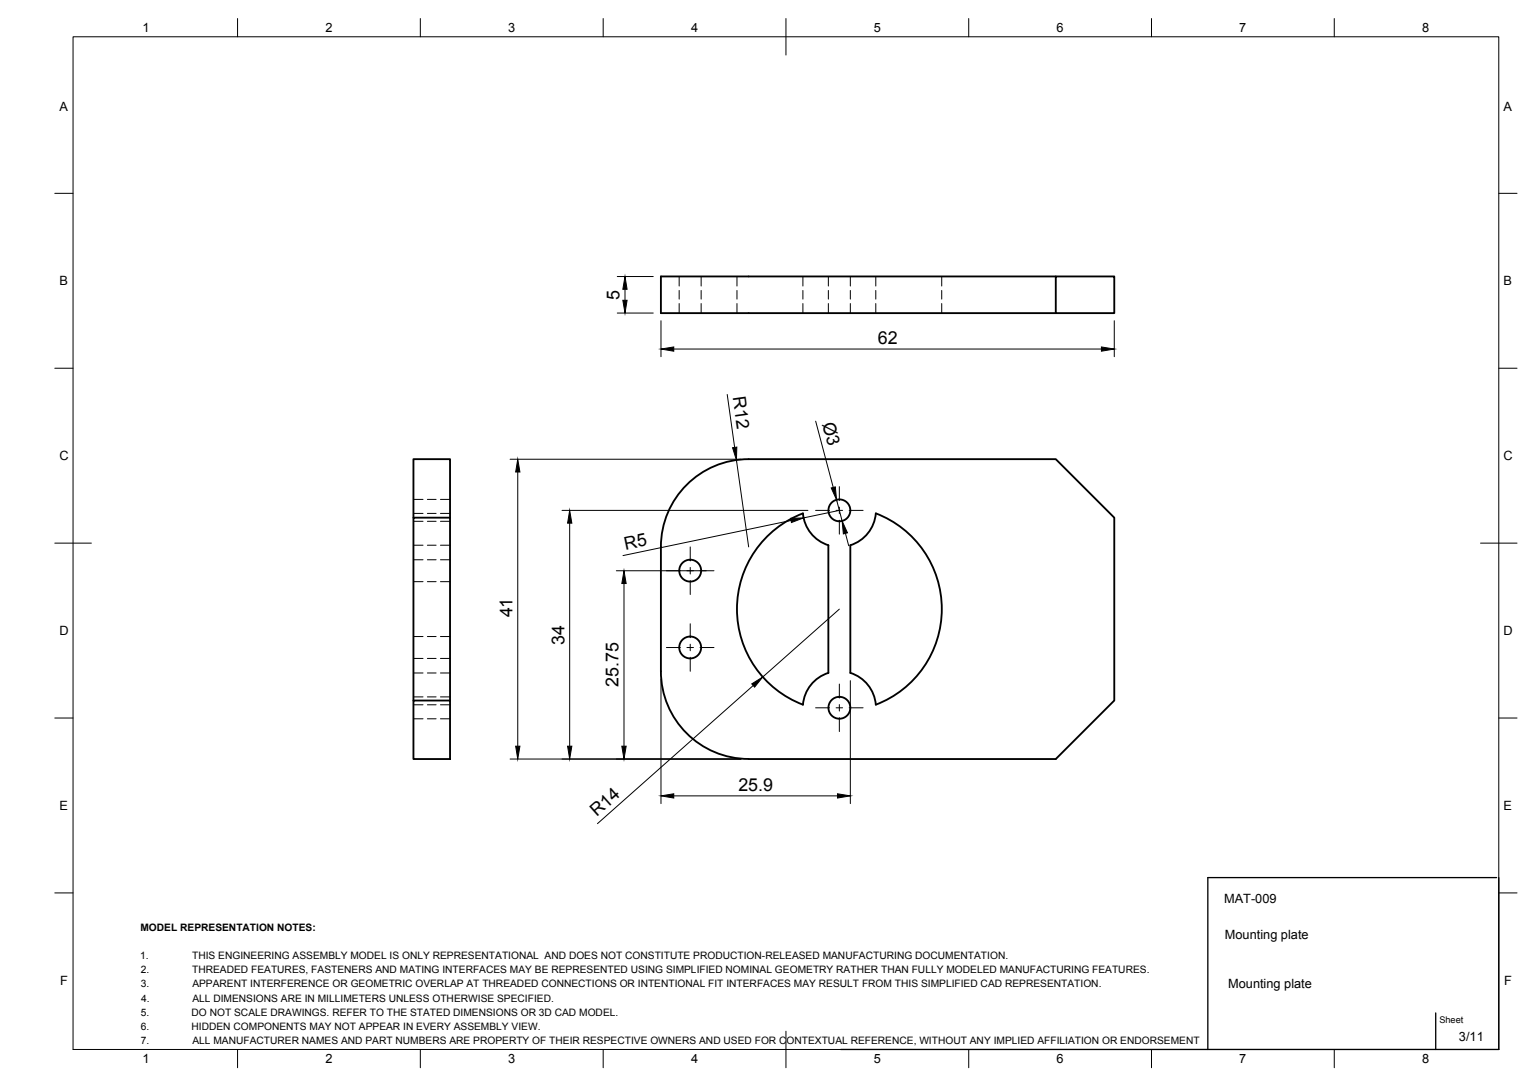
ISO-10303-21;
HEADER;
/* Generated by software containing ST-Developer
 * from STEP Tools, Inc. (www.steptools.com) 
 */

FILE_DESCRIPTION(
/* description */ ('STEP AP214'),
/* implementation_level */ '2;1');

FILE_NAME(
/* name */ 'Mounting Plate.step',
/* time_stamp */ '2026-11-14T05:43:09-08:00',
/* author */ (''),
/* organization */ (''),
/* preprocessor_version */ 'ST-DEVELOPER v20.2',
/* originating_system */ 'Autodesk Translation Framework v15.17.0.0',
/* authorisation */ '');

FILE_SCHEMA (('AUTOMOTIVE_DESIGN { 1 0 10303 214 3 1 1 }'));
ENDSEC;

DATA;
#10=MECHANICAL_DESIGN_GEOMETRIC_PRESENTATION_REPRESENTATION('',(#146),#11933);
#128=SHAPE_REPRESENTATION_RELATIONSHIP('SRR','None',#11988,#137);
#137=ADVANCED_BREP_SHAPE_REPRESENTATION('',(#155),#11924);
#146=STYLED_ITEM('',(#12042),#155);
#155=MANIFOLD_SOLID_BREP('Body1',#6643);
#164=FACE_BOUND('',#692,.T.);
#165=FACE_BOUND('',#693,.T.);
#166=FACE_BOUND('',#694,.T.);
#167=FACE_BOUND('',#695,.T.);
#168=FACE_BOUND('',#696,.T.);
#169=FACE_BOUND('',#697,.T.);
#170=FACE_BOUND('',#699,.T.);
#171=FACE_BOUND('',#700,.T.);
#172=FACE_BOUND('',#701,.T.);
#173=FACE_BOUND('',#702,.T.);
#174=FACE_BOUND('',#703,.T.);
#175=FACE_BOUND('',#704,.T.);
#209=PLANE('',#6766);
#210=PLANE('',#6767);
#211=PLANE('',#6768);
#212=PLANE('',#6769);
#213=PLANE('',#6770);
#214=PLANE('',#6777);
#215=PLANE('',#6787);
#216=PLANE('',#6791);
#217=PLANE('',#6792);
#218=PLANE('',#6795);
#319=FACE_OUTER_BOUND('',#673,.T.);
#320=FACE_OUTER_BOUND('',#674,.T.);
#321=FACE_OUTER_BOUND('',#675,.T.);
#322=FACE_OUTER_BOUND('',#676,.T.);
#323=FACE_OUTER_BOUND('',#677,.T.);
#324=FACE_OUTER_BOUND('',#678,.T.);
#325=FACE_OUTER_BOUND('',#679,.T.);
#326=FACE_OUTER_BOUND('',#680,.T.);
#327=FACE_OUTER_BOUND('',#681,.T.);
#328=FACE_OUTER_BOUND('',#682,.T.);
#329=FACE_OUTER_BOUND('',#683,.T.);
#330=FACE_OUTER_BOUND('',#684,.T.);
#331=FACE_OUTER_BOUND('',#685,.T.);
#332=FACE_OUTER_BOUND('',#686,.T.);
#333=FACE_OUTER_BOUND('',#687,.T.);
#334=FACE_OUTER_BOUND('',#688,.T.);
#335=FACE_OUTER_BOUND('',#689,.T.);
#336=FACE_OUTER_BOUND('',#690,.T.);
#337=FACE_OUTER_BOUND('',#691,.T.);
#338=FACE_OUTER_BOUND('',#698,.T.);
#339=FACE_OUTER_BOUND('',#705,.T.);
#340=FACE_OUTER_BOUND('',#706,.T.);
#673=EDGE_LOOP('',(#4112,#4113,#4114,#4115));
#674=EDGE_LOOP('',(#4116,#4117,#4118,#4119));
#675=EDGE_LOOP('',(#4120,#4121,#4122,#4123));
#676=EDGE_LOOP('',(#4124,#4125,#4126,#4127));
#677=EDGE_LOOP('',(#4128,#4129,#4130,#4131));
#678=EDGE_LOOP('',(#4132,#4133,#4134,#4135));
#679=EDGE_LOOP('',(#4136,#4137,#4138,#4139));
#680=EDGE_LOOP('',(#4140,#4141,#4142,#4143));
#681=EDGE_LOOP('',(#4144,#4145,#4146,#4147));
#682=EDGE_LOOP('',(#4148,#4149,#4150,#4151));
#683=EDGE_LOOP('',(#4152,#4153,#4154,#4155));
#684=EDGE_LOOP('',(#4156,#4157,#4158,#4159));
#685=EDGE_LOOP('',(#4160,#4161,#4162,#4163));
#686=EDGE_LOOP('',(#4164,#4165,#4166,#4167));
#687=EDGE_LOOP('',(#4168,#4169,#4170,#4171));
#688=EDGE_LOOP('',(#4172,#4173,#4174,#4175));
#689=EDGE_LOOP('',(#4176,#4177,#4178,#4179));
#690=EDGE_LOOP('',(#4180,#4181,#4182,#4183));
#691=EDGE_LOOP('',(#4184,#4185,#4186,#4187,#4188,#4189,#4190,#4191));
#692=EDGE_LOOP('',(#4192));
#693=EDGE_LOOP('',(#4193));
#694=EDGE_LOOP('',(#4194));
#695=EDGE_LOOP('',(#4195));
#696=EDGE_LOOP('',(#4196,#4197,#4198,#4199));
#697=EDGE_LOOP('',(#4200,#4201,#4202,#4203));
#698=EDGE_LOOP('',(#4204,#4205,#4206,#4207,#4208,#4209,#4210,#4211));
#699=EDGE_LOOP('',(#4212));
#700=EDGE_LOOP('',(#4213));
#701=EDGE_LOOP('',(#4214));
#702=EDGE_LOOP('',(#4215));
#703=EDGE_LOOP('',(#4216,#4217,#4218,#4219));
#704=EDGE_LOOP('',(#4220,#4221,#4222,#4223));
#705=EDGE_LOOP('',(#4224,#4225,#4226,#4227));
#706=EDGE_LOOP('',(#4228,#4229,#4230,#4231));
#1072=LINE('',#9914,#1534);
#1073=LINE('',#9920,#1535);
#1074=LINE('',#9926,#1536);
#1075=LINE('',#9932,#1537);
#1076=LINE('',#9937,#1538);
#1077=LINE('',#9939,#1539);
#1078=LINE('',#9941,#1540);
#1079=LINE('',#9942,#1541);
#1080=LINE('',#9945,#1542);
#1081=LINE('',#9947,#1543);
#1082=LINE('',#9948,#1544);
#1083=LINE('',#9951,#1545);
#1084=LINE('',#9953,#1546);
#1085=LINE('',#9954,#1547);
#1086=LINE('',#9957,#1548);
#1087=LINE('',#9959,#1549);
#1088=LINE('',#9960,#1550);
#1089=LINE('',#9964,#1551);
#1090=LINE('',#9966,#1552);
#1091=LINE('',#9968,#1553);
#1092=LINE('',#9969,#1554);
#1093=LINE('',#9975,#1555);
#1094=LINE('',#9978,#1556);
#1095=LINE('',#9983,#1557);
#1096=LINE('',#9987,#1558);
#1097=LINE('',#9989,#1559);
#1098=LINE('',#9990,#1560);
#1099=LINE('',#9996,#1561);
#1100=LINE('',#9999,#1562);
#1101=LINE('',#10004,#1563);
#1102=LINE('',#10010,#1564);
#1103=LINE('',#10014,#1565);
#1104=LINE('',#10016,#1566);
#1105=LINE('',#10017,#1567);
#1106=LINE('',#10022,#1568);
#1107=LINE('',#10023,#1569);
#1534=VECTOR('',#7658,1.5);
#1535=VECTOR('',#7665,1.5);
#1536=VECTOR('',#7672,1.5);
#1537=VECTOR('',#7679,1.5);
#1538=VECTOR('',#7684,1000.);
#1539=VECTOR('',#7685,1000.);
#1540=VECTOR('',#7686,1000.);
#1541=VECTOR('',#7687,1000.);
#1542=VECTOR('',#7690,1000.);
#1543=VECTOR('',#7691,1000.);
#1544=VECTOR('',#7692,1000.);
#1545=VECTOR('',#7695,1000.);
#1546=VECTOR('',#7696,1000.);
#1547=VECTOR('',#7697,1000.);
#1548=VECTOR('',#7700,1000.);
#1549=VECTOR('',#7701,1000.);
#1550=VECTOR('',#7702,1000.);
#1551=VECTOR('',#7705,1000.);
#1552=VECTOR('',#7706,1000.);
#1553=VECTOR('',#7707,1000.);
#1554=VECTOR('',#7708,1000.);
#1555=VECTOR('',#7713,1000.);
#1556=VECTOR('',#7716,1000.);
#1557=VECTOR('',#7721,1000.);
#1558=VECTOR('',#7726,1000.);
#1559=VECTOR('',#7727,1000.);
#1560=VECTOR('',#7728,1000.);
#1561=VECTOR('',#7733,1000.);
#1562=VECTOR('',#7736,1000.);
#1563=VECTOR('',#7741,1000.);
#1564=VECTOR('',#7748,1000.);
#1565=VECTOR('',#7753,1000.);
#1566=VECTOR('',#7754,1000.);
#1567=VECTOR('',#7755,1000.);
#1568=VECTOR('',#7764,1000.);
#1569=VECTOR('',#7765,1000.);
#1996=CIRCLE('',#6755,1.5);
#1997=CIRCLE('',#6756,1.5);
#1998=CIRCLE('',#6758,1.5);
#1999=CIRCLE('',#6759,1.5);
#2000=CIRCLE('',#6761,1.5);
#2001=CIRCLE('',#6762,1.5);
#2002=CIRCLE('',#6764,1.5);
#2003=CIRCLE('',#6765,1.5);
#2004=CIRCLE('',#6772,14.);
#2005=CIRCLE('',#6773,14.);
#2006=CIRCLE('',#6775,5.);
#2007=CIRCLE('',#6776,5.);
#2008=CIRCLE('',#6779,5.);
#2009=CIRCLE('',#6780,5.);
#2010=CIRCLE('',#6782,14.);
#2011=CIRCLE('',#6783,14.);
#2012=CIRCLE('',#6785,5.);
#2013=CIRCLE('',#6786,5.);
#2014=CIRCLE('',#6789,5.);
#2015=CIRCLE('',#6790,5.);
#2016=CIRCLE('',#6793,12.);
#2017=CIRCLE('',#6794,12.);
#2018=CIRCLE('',#6796,12.);
#2019=CIRCLE('',#6797,12.);
#2501=VERTEX_POINT('',#9911);
#2502=VERTEX_POINT('',#9913);
#2503=VERTEX_POINT('',#9917);
#2504=VERTEX_POINT('',#9919);
#2505=VERTEX_POINT('',#9923);
#2506=VERTEX_POINT('',#9925);
#2507=VERTEX_POINT('',#9929);
#2508=VERTEX_POINT('',#9931);
#2509=VERTEX_POINT('',#9935);
#2510=VERTEX_POINT('',#9936);
#2511=VERTEX_POINT('',#9938);
#2512=VERTEX_POINT('',#9940);
#2513=VERTEX_POINT('',#9944);
#2514=VERTEX_POINT('',#9946);
#2515=VERTEX_POINT('',#9950);
#2516=VERTEX_POINT('',#9952);
#2517=VERTEX_POINT('',#9956);
#2518=VERTEX_POINT('',#9958);
#2519=VERTEX_POINT('',#9962);
#2520=VERTEX_POINT('',#9963);
#2521=VERTEX_POINT('',#9965);
#2522=VERTEX_POINT('',#9967);
#2523=VERTEX_POINT('',#9971);
#2524=VERTEX_POINT('',#9972);
#2525=VERTEX_POINT('',#9974);
#2526=VERTEX_POINT('',#9976);
#2527=VERTEX_POINT('',#9980);
#2528=VERTEX_POINT('',#9982);
#2529=VERTEX_POINT('',#9986);
#2530=VERTEX_POINT('',#9988);
#2531=VERTEX_POINT('',#9992);
#2532=VERTEX_POINT('',#9993);
#2533=VERTEX_POINT('',#9995);
#2534=VERTEX_POINT('',#9997);
#2535=VERTEX_POINT('',#10001);
#2536=VERTEX_POINT('',#10003);
#2537=VERTEX_POINT('',#10007);
#2538=VERTEX_POINT('',#10009);
#2539=VERTEX_POINT('',#10013);
#2540=VERTEX_POINT('',#10015);
#3145=EDGE_CURVE('',#2501,#2501,#1996,.T.);
#3146=EDGE_CURVE('',#2501,#2502,#1072,.T.);
#3147=EDGE_CURVE('',#2502,#2502,#1997,.T.);
#3148=EDGE_CURVE('',#2503,#2503,#1998,.T.);
#3149=EDGE_CURVE('',#2503,#2504,#1073,.T.);
#3150=EDGE_CURVE('',#2504,#2504,#1999,.T.);
#3151=EDGE_CURVE('',#2505,#2505,#2000,.T.);
#3152=EDGE_CURVE('',#2505,#2506,#1074,.T.);
#3153=EDGE_CURVE('',#2506,#2506,#2001,.T.);
#3154=EDGE_CURVE('',#2507,#2507,#2002,.T.);
#3155=EDGE_CURVE('',#2507,#2508,#1075,.T.);
#3156=EDGE_CURVE('',#2508,#2508,#2003,.T.);
#3157=EDGE_CURVE('',#2509,#2510,#1076,.T.);
#3158=EDGE_CURVE('',#2511,#2510,#1077,.T.);
#3159=EDGE_CURVE('',#2512,#2511,#1078,.T.);
#3160=EDGE_CURVE('',#2512,#2509,#1079,.T.);
#3161=EDGE_CURVE('',#2510,#2513,#1080,.T.);
#3162=EDGE_CURVE('',#2514,#2513,#1081,.T.);
#3163=EDGE_CURVE('',#2511,#2514,#1082,.T.);
#3164=EDGE_CURVE('',#2515,#2513,#1083,.T.);
#3165=EDGE_CURVE('',#2516,#2515,#1084,.T.);
#3166=EDGE_CURVE('',#2516,#2514,#1085,.T.);
#3167=EDGE_CURVE('',#2515,#2517,#1086,.T.);
#3168=EDGE_CURVE('',#2517,#2518,#1087,.T.);
#3169=EDGE_CURVE('',#2516,#2518,#1088,.T.);
#3170=EDGE_CURVE('',#2519,#2520,#1089,.T.);
#3171=EDGE_CURVE('',#2519,#2521,#1090,.T.);
#3172=EDGE_CURVE('',#2521,#2522,#1091,.T.);
#3173=EDGE_CURVE('',#2522,#2520,#1092,.T.);
#3174=EDGE_CURVE('',#2523,#2524,#2004,.T.);
#3175=EDGE_CURVE('',#2525,#2523,#1093,.T.);
#3176=EDGE_CURVE('',#2525,#2526,#2005,.T.);
#3177=EDGE_CURVE('',#2526,#2524,#1094,.T.);
#3178=EDGE_CURVE('',#2527,#2523,#2006,.T.);
#3179=EDGE_CURVE('',#2528,#2527,#1095,.T.);
#3180=EDGE_CURVE('',#2528,#2525,#2007,.T.);
#3181=EDGE_CURVE('',#2529,#2527,#1096,.T.);
#3182=EDGE_CURVE('',#2530,#2529,#1097,.T.);
#3183=EDGE_CURVE('',#2530,#2528,#1098,.T.);
#3184=EDGE_CURVE('',#2531,#2532,#2008,.T.);
#3185=EDGE_CURVE('',#2533,#2531,#1099,.T.);
#3186=EDGE_CURVE('',#2533,#2534,#2009,.T.);
#3187=EDGE_CURVE('',#2534,#2532,#1100,.T.);
#3188=EDGE_CURVE('',#2535,#2531,#2010,.T.);
#3189=EDGE_CURVE('',#2536,#2535,#1101,.T.);
#3190=EDGE_CURVE('',#2536,#2533,#2011,.T.);
#3191=EDGE_CURVE('',#2535,#2537,#2012,.T.);
#3192=EDGE_CURVE('',#2538,#2537,#1102,.T.);
#3193=EDGE_CURVE('',#2536,#2538,#2013,.T.);
#3194=EDGE_CURVE('',#2539,#2512,#1103,.T.);
#3195=EDGE_CURVE('',#2539,#2540,#1104,.T.);
#3196=EDGE_CURVE('',#2540,#2509,#1105,.T.);
#3197=EDGE_CURVE('',#2529,#2524,#2014,.T.);
#3198=EDGE_CURVE('',#2530,#2526,#2015,.T.);
#3199=EDGE_CURVE('',#2537,#2532,#1106,.T.);
#3200=EDGE_CURVE('',#2538,#2534,#1107,.T.);
#3201=EDGE_CURVE('',#2518,#2519,#2016,.T.);
#3202=EDGE_CURVE('',#2520,#2539,#2017,.T.);
#3203=EDGE_CURVE('',#2521,#2517,#2018,.T.);
#3204=EDGE_CURVE('',#2540,#2522,#2019,.T.);
#4112=ORIENTED_EDGE('',*,*,#3145,.F.);
#4113=ORIENTED_EDGE('',*,*,#3146,.T.);
#4114=ORIENTED_EDGE('',*,*,#3147,.T.);
#4115=ORIENTED_EDGE('',*,*,#3146,.F.);
#4116=ORIENTED_EDGE('',*,*,#3148,.T.);
#4117=ORIENTED_EDGE('',*,*,#3149,.T.);
#4118=ORIENTED_EDGE('',*,*,#3150,.F.);
#4119=ORIENTED_EDGE('',*,*,#3149,.F.);
#4120=ORIENTED_EDGE('',*,*,#3151,.T.);
#4121=ORIENTED_EDGE('',*,*,#3152,.T.);
#4122=ORIENTED_EDGE('',*,*,#3153,.F.);
#4123=ORIENTED_EDGE('',*,*,#3152,.F.);
#4124=ORIENTED_EDGE('',*,*,#3154,.T.);
#4125=ORIENTED_EDGE('',*,*,#3155,.T.);
#4126=ORIENTED_EDGE('',*,*,#3156,.F.);
#4127=ORIENTED_EDGE('',*,*,#3155,.F.);
#4128=ORIENTED_EDGE('',*,*,#3157,.T.);
#4129=ORIENTED_EDGE('',*,*,#3158,.F.);
#4130=ORIENTED_EDGE('',*,*,#3159,.F.);
#4131=ORIENTED_EDGE('',*,*,#3160,.T.);
#4132=ORIENTED_EDGE('',*,*,#3161,.T.);
#4133=ORIENTED_EDGE('',*,*,#3162,.F.);
#4134=ORIENTED_EDGE('',*,*,#3163,.F.);
#4135=ORIENTED_EDGE('',*,*,#3158,.T.);
#4136=ORIENTED_EDGE('',*,*,#3164,.F.);
#4137=ORIENTED_EDGE('',*,*,#3165,.F.);
#4138=ORIENTED_EDGE('',*,*,#3166,.T.);
#4139=ORIENTED_EDGE('',*,*,#3162,.T.);
#4140=ORIENTED_EDGE('',*,*,#3167,.T.);
#4141=ORIENTED_EDGE('',*,*,#3168,.T.);
#4142=ORIENTED_EDGE('',*,*,#3169,.F.);
#4143=ORIENTED_EDGE('',*,*,#3165,.T.);
#4144=ORIENTED_EDGE('',*,*,#3170,.F.);
#4145=ORIENTED_EDGE('',*,*,#3171,.T.);
#4146=ORIENTED_EDGE('',*,*,#3172,.T.);
#4147=ORIENTED_EDGE('',*,*,#3173,.T.);
#4148=ORIENTED_EDGE('',*,*,#3174,.F.);
#4149=ORIENTED_EDGE('',*,*,#3175,.F.);
#4150=ORIENTED_EDGE('',*,*,#3176,.T.);
#4151=ORIENTED_EDGE('',*,*,#3177,.T.);
#4152=ORIENTED_EDGE('',*,*,#3178,.F.);
#4153=ORIENTED_EDGE('',*,*,#3179,.F.);
#4154=ORIENTED_EDGE('',*,*,#3180,.T.);
#4155=ORIENTED_EDGE('',*,*,#3175,.T.);
#4156=ORIENTED_EDGE('',*,*,#3181,.F.);
#4157=ORIENTED_EDGE('',*,*,#3182,.F.);
#4158=ORIENTED_EDGE('',*,*,#3183,.T.);
#4159=ORIENTED_EDGE('',*,*,#3179,.T.);
#4160=ORIENTED_EDGE('',*,*,#3184,.F.);
#4161=ORIENTED_EDGE('',*,*,#3185,.F.);
#4162=ORIENTED_EDGE('',*,*,#3186,.T.);
#4163=ORIENTED_EDGE('',*,*,#3187,.T.);
#4164=ORIENTED_EDGE('',*,*,#3188,.F.);
#4165=ORIENTED_EDGE('',*,*,#3189,.F.);
#4166=ORIENTED_EDGE('',*,*,#3190,.T.);
#4167=ORIENTED_EDGE('',*,*,#3185,.T.);
#4168=ORIENTED_EDGE('',*,*,#3191,.T.);
#4169=ORIENTED_EDGE('',*,*,#3192,.F.);
#4170=ORIENTED_EDGE('',*,*,#3193,.F.);
#4171=ORIENTED_EDGE('',*,*,#3189,.T.);
#4172=ORIENTED_EDGE('',*,*,#3194,.F.);
#4173=ORIENTED_EDGE('',*,*,#3195,.T.);
#4174=ORIENTED_EDGE('',*,*,#3196,.T.);
#4175=ORIENTED_EDGE('',*,*,#3160,.F.);
#4176=ORIENTED_EDGE('',*,*,#3197,.T.);
#4177=ORIENTED_EDGE('',*,*,#3177,.F.);
#4178=ORIENTED_EDGE('',*,*,#3198,.F.);
#4179=ORIENTED_EDGE('',*,*,#3182,.T.);
#4180=ORIENTED_EDGE('',*,*,#3199,.T.);
#4181=ORIENTED_EDGE('',*,*,#3187,.F.);
#4182=ORIENTED_EDGE('',*,*,#3200,.F.);
#4183=ORIENTED_EDGE('',*,*,#3192,.T.);
#4184=ORIENTED_EDGE('',*,*,#3169,.T.);
#4185=ORIENTED_EDGE('',*,*,#3201,.T.);
#4186=ORIENTED_EDGE('',*,*,#3170,.T.);
#4187=ORIENTED_EDGE('',*,*,#3202,.T.);
#4188=ORIENTED_EDGE('',*,*,#3194,.T.);
#4189=ORIENTED_EDGE('',*,*,#3159,.T.);
#4190=ORIENTED_EDGE('',*,*,#3163,.T.);
#4191=ORIENTED_EDGE('',*,*,#3166,.F.);
#4192=ORIENTED_EDGE('',*,*,#3154,.F.);
#4193=ORIENTED_EDGE('',*,*,#3145,.T.);
#4194=ORIENTED_EDGE('',*,*,#3148,.F.);
#4195=ORIENTED_EDGE('',*,*,#3151,.F.);
#4196=ORIENTED_EDGE('',*,*,#3186,.F.);
#4197=ORIENTED_EDGE('',*,*,#3190,.F.);
#4198=ORIENTED_EDGE('',*,*,#3193,.T.);
#4199=ORIENTED_EDGE('',*,*,#3200,.T.);
#4200=ORIENTED_EDGE('',*,*,#3176,.F.);
#4201=ORIENTED_EDGE('',*,*,#3180,.F.);
#4202=ORIENTED_EDGE('',*,*,#3183,.F.);
#4203=ORIENTED_EDGE('',*,*,#3198,.T.);
#4204=ORIENTED_EDGE('',*,*,#3172,.F.);
#4205=ORIENTED_EDGE('',*,*,#3203,.T.);
#4206=ORIENTED_EDGE('',*,*,#3167,.F.);
#4207=ORIENTED_EDGE('',*,*,#3164,.T.);
#4208=ORIENTED_EDGE('',*,*,#3161,.F.);
#4209=ORIENTED_EDGE('',*,*,#3157,.F.);
#4210=ORIENTED_EDGE('',*,*,#3196,.F.);
#4211=ORIENTED_EDGE('',*,*,#3204,.T.);
#4212=ORIENTED_EDGE('',*,*,#3156,.T.);
#4213=ORIENTED_EDGE('',*,*,#3147,.F.);
#4214=ORIENTED_EDGE('',*,*,#3150,.T.);
#4215=ORIENTED_EDGE('',*,*,#3153,.T.);
#4216=ORIENTED_EDGE('',*,*,#3184,.T.);
#4217=ORIENTED_EDGE('',*,*,#3199,.F.);
#4218=ORIENTED_EDGE('',*,*,#3191,.F.);
#4219=ORIENTED_EDGE('',*,*,#3188,.T.);
#4220=ORIENTED_EDGE('',*,*,#3174,.T.);
#4221=ORIENTED_EDGE('',*,*,#3197,.F.);
#4222=ORIENTED_EDGE('',*,*,#3181,.T.);
#4223=ORIENTED_EDGE('',*,*,#3178,.T.);
#4224=ORIENTED_EDGE('',*,*,#3201,.F.);
#4225=ORIENTED_EDGE('',*,*,#3168,.F.);
#4226=ORIENTED_EDGE('',*,*,#3203,.F.);
#4227=ORIENTED_EDGE('',*,*,#3171,.F.);
#4228=ORIENTED_EDGE('',*,*,#3202,.F.);
#4229=ORIENTED_EDGE('',*,*,#3173,.F.);
#4230=ORIENTED_EDGE('',*,*,#3204,.F.);
#4231=ORIENTED_EDGE('',*,*,#3195,.F.);
#6046=CYLINDRICAL_SURFACE('',#6754,1.5);
#6047=CYLINDRICAL_SURFACE('',#6757,1.5);
#6048=CYLINDRICAL_SURFACE('',#6760,1.5);
#6049=CYLINDRICAL_SURFACE('',#6763,1.5);
#6050=CYLINDRICAL_SURFACE('',#6771,14.);
#6051=CYLINDRICAL_SURFACE('',#6774,5.);
#6052=CYLINDRICAL_SURFACE('',#6778,5.);
#6053=CYLINDRICAL_SURFACE('',#6781,14.);
#6054=CYLINDRICAL_SURFACE('',#6784,5.);
#6055=CYLINDRICAL_SURFACE('',#6788,5.);
#6056=CYLINDRICAL_SURFACE('',#6798,12.);
#6057=CYLINDRICAL_SURFACE('',#6799,12.);
#6289=ADVANCED_FACE('',(#319),#6046,.F.);
#6290=ADVANCED_FACE('',(#320),#6047,.F.);
#6291=ADVANCED_FACE('',(#321),#6048,.F.);
#6292=ADVANCED_FACE('',(#322),#6049,.F.);
#6293=ADVANCED_FACE('',(#323),#209,.F.);
#6294=ADVANCED_FACE('',(#324),#210,.F.);
#6295=ADVANCED_FACE('',(#325),#211,.T.);
#6296=ADVANCED_FACE('',(#326),#212,.F.);
#6297=ADVANCED_FACE('',(#327),#213,.F.);
#6298=ADVANCED_FACE('',(#328),#6050,.F.);
#6299=ADVANCED_FACE('',(#329),#6051,.T.);
#6300=ADVANCED_FACE('',(#330),#214,.T.);
#6301=ADVANCED_FACE('',(#331),#6052,.T.);
#6302=ADVANCED_FACE('',(#332),#6053,.F.);
#6303=ADVANCED_FACE('',(#333),#6054,.T.);
#6304=ADVANCED_FACE('',(#334),#215,.F.);
#6305=ADVANCED_FACE('',(#335),#6055,.T.);
#6306=ADVANCED_FACE('',(#336),#216,.F.);
#6307=ADVANCED_FACE('',(#337,#164,#165,#166,#167,#168,#169),#217,.T.);
#6308=ADVANCED_FACE('',(#338,#170,#171,#172,#173,#174,#175),#218,.F.);
#6309=ADVANCED_FACE('',(#339),#6056,.T.);
#6310=ADVANCED_FACE('',(#340),#6057,.T.);
#6643=CLOSED_SHELL('',(#6289,#6290,#6291,#6292,#6293,#6294,#6295,#6296,
#6297,#6298,#6299,#6300,#6301,#6302,#6303,#6304,#6305,#6306,#6307,#6308,
#6309,#6310));
#6753=AXIS2_PLACEMENT_3D('',#9909,#7652,#7653);
#6754=AXIS2_PLACEMENT_3D('',#9910,#7654,#7655);
#6755=AXIS2_PLACEMENT_3D('',#9912,#7656,#7657);
#6756=AXIS2_PLACEMENT_3D('',#9915,#7659,#7660);
#6757=AXIS2_PLACEMENT_3D('',#9916,#7661,#7662);
#6758=AXIS2_PLACEMENT_3D('',#9918,#7663,#7664);
#6759=AXIS2_PLACEMENT_3D('',#9921,#7666,#7667);
#6760=AXIS2_PLACEMENT_3D('',#9922,#7668,#7669);
#6761=AXIS2_PLACEMENT_3D('',#9924,#7670,#7671);
#6762=AXIS2_PLACEMENT_3D('',#9927,#7673,#7674);
#6763=AXIS2_PLACEMENT_3D('',#9928,#7675,#7676);
#6764=AXIS2_PLACEMENT_3D('',#9930,#7677,#7678);
#6765=AXIS2_PLACEMENT_3D('',#9933,#7680,#7681);
#6766=AXIS2_PLACEMENT_3D('',#9934,#7682,#7683);
#6767=AXIS2_PLACEMENT_3D('',#9943,#7688,#7689);
#6768=AXIS2_PLACEMENT_3D('',#9949,#7693,#7694);
#6769=AXIS2_PLACEMENT_3D('',#9955,#7698,#7699);
#6770=AXIS2_PLACEMENT_3D('',#9961,#7703,#7704);
#6771=AXIS2_PLACEMENT_3D('',#9970,#7709,#7710);
#6772=AXIS2_PLACEMENT_3D('',#9973,#7711,#7712);
#6773=AXIS2_PLACEMENT_3D('',#9977,#7714,#7715);
#6774=AXIS2_PLACEMENT_3D('',#9979,#7717,#7718);
#6775=AXIS2_PLACEMENT_3D('',#9981,#7719,#7720);
#6776=AXIS2_PLACEMENT_3D('',#9984,#7722,#7723);
#6777=AXIS2_PLACEMENT_3D('',#9985,#7724,#7725);
#6778=AXIS2_PLACEMENT_3D('',#9991,#7729,#7730);
#6779=AXIS2_PLACEMENT_3D('',#9994,#7731,#7732);
#6780=AXIS2_PLACEMENT_3D('',#9998,#7734,#7735);
#6781=AXIS2_PLACEMENT_3D('',#10000,#7737,#7738);
#6782=AXIS2_PLACEMENT_3D('',#10002,#7739,#7740);
#6783=AXIS2_PLACEMENT_3D('',#10005,#7742,#7743);
#6784=AXIS2_PLACEMENT_3D('',#10006,#7744,#7745);
#6785=AXIS2_PLACEMENT_3D('',#10008,#7746,#7747);
#6786=AXIS2_PLACEMENT_3D('',#10011,#7749,#7750);
#6787=AXIS2_PLACEMENT_3D('',#10012,#7751,#7752);
#6788=AXIS2_PLACEMENT_3D('',#10018,#7756,#7757);
#6789=AXIS2_PLACEMENT_3D('',#10019,#7758,#7759);
#6790=AXIS2_PLACEMENT_3D('',#10020,#7760,#7761);
#6791=AXIS2_PLACEMENT_3D('',#10021,#7762,#7763);
#6792=AXIS2_PLACEMENT_3D('',#10024,#7766,#7767);
#6793=AXIS2_PLACEMENT_3D('',#10025,#7768,#7769);
#6794=AXIS2_PLACEMENT_3D('',#10026,#7770,#7771);
#6795=AXIS2_PLACEMENT_3D('',#10027,#7772,#7773);
#6796=AXIS2_PLACEMENT_3D('',#10028,#7774,#7775);
#6797=AXIS2_PLACEMENT_3D('',#10029,#7776,#7777);
#6798=AXIS2_PLACEMENT_3D('',#10030,#7778,#7779);
#6799=AXIS2_PLACEMENT_3D('',#10031,#7780,#7781);
#7652=DIRECTION('axis',(0.,0.,1.));
#7653=DIRECTION('refdir',(1.,0.,0.));
#7654=DIRECTION('center_axis',(0.,0.,-1.));
#7655=DIRECTION('ref_axis',(-1.,0.,0.));
#7656=DIRECTION('center_axis',(0.,0.,-1.));
#7657=DIRECTION('ref_axis',(1.,0.,0.));
#7658=DIRECTION('',(0.,0.,-1.));
#7659=DIRECTION('center_axis',(0.,0.,-1.));
#7660=DIRECTION('ref_axis',(1.,0.,0.));
#7661=DIRECTION('center_axis',(0.,0.,-1.));
#7662=DIRECTION('ref_axis',(-1.,0.,0.));
#7663=DIRECTION('center_axis',(0.,0.,1.));
#7664=DIRECTION('ref_axis',(1.,0.,0.));
#7665=DIRECTION('',(0.,0.,-1.));
#7666=DIRECTION('center_axis',(0.,0.,1.));
#7667=DIRECTION('ref_axis',(1.,0.,0.));
#7668=DIRECTION('center_axis',(0.,0.,-1.));
#7669=DIRECTION('ref_axis',(-1.,0.,0.));
#7670=DIRECTION('center_axis',(0.,0.,1.));
#7671=DIRECTION('ref_axis',(1.,0.,0.));
#7672=DIRECTION('',(0.,0.,-1.));
#7673=DIRECTION('center_axis',(0.,0.,1.));
#7674=DIRECTION('ref_axis',(1.,0.,0.));
#7675=DIRECTION('center_axis',(0.,0.,-1.));
#7676=DIRECTION('ref_axis',(-1.,0.,0.));
#7677=DIRECTION('center_axis',(0.,0.,1.));
#7678=DIRECTION('ref_axis',(1.,0.,0.));
#7679=DIRECTION('',(0.,0.,-1.));
#7680=DIRECTION('center_axis',(0.,0.,1.));
#7681=DIRECTION('ref_axis',(1.,0.,0.));
#7682=DIRECTION('center_axis',(0.707106781186548,0.707106781186548,0.));
#7683=DIRECTION('ref_axis',(-0.707106781186548,0.707106781186548,0.));
#7684=DIRECTION('',(0.707106781186547,-0.707106781186547,0.));
#7685=DIRECTION('',(0.,0.,-1.));
#7686=DIRECTION('',(0.707106781186547,-0.707106781186547,0.));
#7687=DIRECTION('',(0.,0.,-1.));
#7688=DIRECTION('center_axis',(0.,1.,0.));
#7689=DIRECTION('ref_axis',(0.,0.,1.));
#7690=DIRECTION('',(1.,0.,0.));
#7691=DIRECTION('',(0.,0.,-1.));
#7692=DIRECTION('',(1.,0.,0.));
#7693=DIRECTION('center_axis',(0.707106781186548,-0.707106781186548,0.));
#7694=DIRECTION('ref_axis',(0.707106781186548,0.707106781186548,0.));
#7695=DIRECTION('',(-0.707106781186547,-0.707106781186547,0.));
#7696=DIRECTION('',(0.,0.,-1.));
#7697=DIRECTION('',(-0.707106781186547,-0.707106781186547,0.));
#7698=DIRECTION('center_axis',(-1.,2.56996070515082E-16,0.));
#7699=DIRECTION('ref_axis',(-2.56996070515082E-16,-1.,0.));
#7700=DIRECTION('',(2.56996070515082E-16,1.,0.));
#7701=DIRECTION('',(0.,0.,1.));
#7702=DIRECTION('',(2.56996070515082E-16,1.,0.));
#7703=DIRECTION('center_axis',(0.,-1.,0.));
#7704=DIRECTION('ref_axis',(0.,0.,-1.));
#7705=DIRECTION('',(-1.,0.,0.));
#7706=DIRECTION('',(0.,0.,-1.));
#7707=DIRECTION('',(-1.,0.,0.));
#7708=DIRECTION('',(0.,0.,1.));
#7709=DIRECTION('center_axis',(0.,0.,-1.));
#7710=DIRECTION('ref_axis',(-1.,0.,0.));
#7711=DIRECTION('center_axis',(0.,0.,1.));
#7712=DIRECTION('ref_axis',(1.,0.,0.));
#7713=DIRECTION('',(0.,0.,-1.));
#7714=DIRECTION('center_axis',(0.,0.,1.));
#7715=DIRECTION('ref_axis',(1.,0.,0.));
#7716=DIRECTION('',(0.,0.,-1.));
#7717=DIRECTION('center_axis',(0.,0.,-1.));
#7718=DIRECTION('ref_axis',(-1.,0.,0.));
#7719=DIRECTION('center_axis',(0.,0.,-1.));
#7720=DIRECTION('ref_axis',(1.,1.77635683940025E-15,0.));
#7721=DIRECTION('',(0.,0.,-1.));
#7722=DIRECTION('center_axis',(0.,0.,-1.));
#7723=DIRECTION('ref_axis',(1.,1.77635683940025E-15,0.));
#7724=DIRECTION('center_axis',(0.,1.,0.));
#7725=DIRECTION('ref_axis',(0.,0.,1.));
#7726=DIRECTION('',(1.,0.,0.));
#7727=DIRECTION('',(0.,0.,-1.));
#7728=DIRECTION('',(1.,0.,0.));
#7729=DIRECTION('center_axis',(0.,0.,-1.));
#7730=DIRECTION('ref_axis',(-1.,0.,0.));
#7731=DIRECTION('center_axis',(0.,0.,-1.));
#7732=DIRECTION('ref_axis',(1.,8.88178419700125E-16,0.));
#7733=DIRECTION('',(0.,0.,-1.));
#7734=DIRECTION('center_axis',(0.,0.,-1.));
#7735=DIRECTION('ref_axis',(1.,8.88178419700125E-16,0.));
#7736=DIRECTION('',(0.,0.,-1.));
#7737=DIRECTION('center_axis',(0.,0.,-1.));
#7738=DIRECTION('ref_axis',(-1.,0.,0.));
#7739=DIRECTION('center_axis',(0.,0.,1.));
#7740=DIRECTION('ref_axis',(1.,0.,0.));
#7741=DIRECTION('',(0.,0.,-1.));
#7742=DIRECTION('center_axis',(0.,0.,1.));
#7743=DIRECTION('ref_axis',(1.,0.,0.));
#7744=DIRECTION('center_axis',(0.,0.,-1.));
#7745=DIRECTION('ref_axis',(-1.,0.,0.));
#7746=DIRECTION('center_axis',(0.,0.,1.));
#7747=DIRECTION('ref_axis',(1.,0.,0.));
#7748=DIRECTION('',(0.,0.,-1.));
#7749=DIRECTION('center_axis',(0.,0.,1.));
#7750=DIRECTION('ref_axis',(1.,0.,0.));
#7751=DIRECTION('center_axis',(1.,1.28498035257541E-16,0.));
#7752=DIRECTION('ref_axis',(-1.28498035257541E-16,1.,0.));
#7753=DIRECTION('',(1.28498035257541E-16,-1.,0.));
#7754=DIRECTION('',(0.,0.,-1.));
#7755=DIRECTION('',(1.28498035257541E-16,-1.,0.));
#7756=DIRECTION('center_axis',(0.,0.,-1.));
#7757=DIRECTION('ref_axis',(-1.,0.,0.));
#7758=DIRECTION('center_axis',(0.,0.,1.));
#7759=DIRECTION('ref_axis',(1.,0.,0.));
#7760=DIRECTION('center_axis',(0.,0.,1.));
#7761=DIRECTION('ref_axis',(1.,0.,0.));
#7762=DIRECTION('center_axis',(0.,1.,0.));
#7763=DIRECTION('ref_axis',(0.,0.,1.));
#7764=DIRECTION('',(1.,0.,0.));
#7765=DIRECTION('',(1.,0.,0.));
#7766=DIRECTION('center_axis',(0.,0.,1.));
#7767=DIRECTION('ref_axis',(1.,0.,0.));
#7768=DIRECTION('center_axis',(0.,0.,1.));
#7769=DIRECTION('ref_axis',(1.,0.,0.));
#7770=DIRECTION('center_axis',(0.,0.,1.));
#7771=DIRECTION('ref_axis',(1.,0.,0.));
#7772=DIRECTION('center_axis',(0.,0.,1.));
#7773=DIRECTION('ref_axis',(1.,0.,0.));
#7774=DIRECTION('center_axis',(0.,0.,-1.));
#7775=DIRECTION('ref_axis',(1.,0.,0.));
#7776=DIRECTION('center_axis',(0.,0.,-1.));
#7777=DIRECTION('ref_axis',(1.,0.,0.));
#7778=DIRECTION('center_axis',(0.,0.,-1.));
#7779=DIRECTION('ref_axis',(-1.,0.,0.));
#7780=DIRECTION('center_axis',(0.,0.,-1.));
#7781=DIRECTION('ref_axis',(-1.,0.,0.));
#9909=CARTESIAN_POINT('',(0.,0.,0.));
#9910=CARTESIAN_POINT('Origin',(13.5,-1.65327317884893E-15,5.));
#9911=CARTESIAN_POINT('',(15.,-1.83697019872103E-15,5.));
#9912=CARTESIAN_POINT('Origin',(13.5,-1.65327317884893E-15,5.));
#9913=CARTESIAN_POINT('',(15.,-1.83697019872103E-15,0.));
#9914=CARTESIAN_POINT('',(15.,-1.83697019872103E-15,5.));
#9915=CARTESIAN_POINT('Origin',(13.5,-1.65327317884893E-15,0.));
#9916=CARTESIAN_POINT('Origin',(-5.24999999999999,20.4,5.));
#9917=CARTESIAN_POINT('',(-3.74999999999999,20.4,5.));
#9918=CARTESIAN_POINT('Origin',(-5.24999999999999,20.4,5.));
#9919=CARTESIAN_POINT('',(-3.74999999999999,20.4,0.));
#9920=CARTESIAN_POINT('',(-3.74999999999999,20.4,5.));
#9921=CARTESIAN_POINT('Origin',(-5.24999999999999,20.4,0.));
#9922=CARTESIAN_POINT('Origin',(5.25000000000001,20.4,5.));
#9923=CARTESIAN_POINT('',(6.75000000000001,20.4,5.));
#9924=CARTESIAN_POINT('Origin',(5.25000000000001,20.4,5.));
#9925=CARTESIAN_POINT('',(6.75000000000001,20.4,0.));
#9926=CARTESIAN_POINT('',(6.75000000000001,20.4,5.));
#9927=CARTESIAN_POINT('Origin',(5.25000000000001,20.4,0.));
#9928=CARTESIAN_POINT('Origin',(-13.5,-1.65327317884893E-15,5.));
#9929=CARTESIAN_POINT('',(-12.,-1.83697019872103E-15,5.));
#9930=CARTESIAN_POINT('Origin',(-13.5,-1.65327317884893E-15,5.));
#9931=CARTESIAN_POINT('',(-12.,-1.83697019872103E-15,0.));
#9932=CARTESIAN_POINT('',(-12.,-1.83697019872103E-15,5.));
#9933=CARTESIAN_POINT('Origin',(-13.5,-1.65327317884893E-15,0.));
#9934=CARTESIAN_POINT('Origin',(-25.05,-25.05,5.));
#9935=CARTESIAN_POINT('',(-20.5,-29.6,0.));
#9936=CARTESIAN_POINT('',(-12.5,-37.6,0.));
#9937=CARTESIAN_POINT('',(-25.05,-25.05,0.));
#9938=CARTESIAN_POINT('',(-12.5,-37.6,5.));
#9939=CARTESIAN_POINT('',(-12.5,-37.6,5.));
#9940=CARTESIAN_POINT('',(-20.5,-29.6,5.));
#9941=CARTESIAN_POINT('',(-25.05,-25.05,5.));
#9942=CARTESIAN_POINT('',(-20.5,-29.6,5.));
#9943=CARTESIAN_POINT('Origin',(0.,-37.6,5.));
#9944=CARTESIAN_POINT('',(12.5,-37.6,0.));
#9945=CARTESIAN_POINT('',(0.,-37.6,0.));
#9946=CARTESIAN_POINT('',(12.5,-37.6,5.));
#9947=CARTESIAN_POINT('',(12.5,-37.6,5.));
#9948=CARTESIAN_POINT('',(0.,-37.6,5.));
#9949=CARTESIAN_POINT('Origin',(25.05,-25.05,5.));
#9950=CARTESIAN_POINT('',(20.5,-29.6,0.));
#9951=CARTESIAN_POINT('',(25.05,-25.05,0.));
#9952=CARTESIAN_POINT('',(20.5,-29.6,5.));
#9953=CARTESIAN_POINT('',(20.5,-29.6,5.));
#9954=CARTESIAN_POINT('',(25.05,-25.05,5.));
#9955=CARTESIAN_POINT('Origin',(20.5,-5.26841944555919E-15,5.));
#9956=CARTESIAN_POINT('',(20.5,12.4,0.));
#9957=CARTESIAN_POINT('',(20.5,-5.26841944555919E-15,0.));
#9958=CARTESIAN_POINT('',(20.5,12.4,5.));
#9959=CARTESIAN_POINT('',(20.5,12.4,5.));
#9960=CARTESIAN_POINT('',(20.5,-5.26841944555919E-15,5.));
#9961=CARTESIAN_POINT('Origin',(0.,24.4,5.));
#9962=CARTESIAN_POINT('',(8.5,24.4,5.));
#9963=CARTESIAN_POINT('',(-8.5,24.4,5.));
#9964=CARTESIAN_POINT('',(0.,24.4,5.));
#9965=CARTESIAN_POINT('',(8.5,24.4,0.));
#9966=CARTESIAN_POINT('',(8.5,24.4,5.));
#9967=CARTESIAN_POINT('',(-8.5,24.4,0.));
#9968=CARTESIAN_POINT('',(0.,24.4,0.));
#9969=CARTESIAN_POINT('',(-8.5,24.4,5.));
#9970=CARTESIAN_POINT('Origin',(0.,0.,5.));
#9971=CARTESIAN_POINT('',(13.0833333333333,4.98260864295891,0.));
#9972=CARTESIAN_POINT('',(-13.0833333333333,4.98260864295891,0.));
#9973=CARTESIAN_POINT('Origin',(0.,0.,0.));
#9974=CARTESIAN_POINT('',(13.0833333333333,4.98260864295891,5.));
#9975=CARTESIAN_POINT('',(13.0833333333333,4.98260864295891,5.));
#9976=CARTESIAN_POINT('',(-13.0833333333333,4.98260864295891,5.));
#9977=CARTESIAN_POINT('Origin',(0.,0.,5.));
#9978=CARTESIAN_POINT('',(-13.0833333333333,4.98260864295891,5.));
#9979=CARTESIAN_POINT('Origin',(13.5,-1.65327317884893E-15,5.));
#9980=CARTESIAN_POINT('',(8.73030399291527,1.5,0.));
#9981=CARTESIAN_POINT('Origin',(13.5,-1.65327317884893E-15,0.));
#9982=CARTESIAN_POINT('',(8.73030399291527,1.5,5.));
#9983=CARTESIAN_POINT('',(8.73030399291527,1.5,5.));
#9984=CARTESIAN_POINT('Origin',(13.5,-1.65327317884893E-15,5.));
#9985=CARTESIAN_POINT('Origin',(0.,1.5,5.));
#9986=CARTESIAN_POINT('',(-8.73030399291527,1.5,0.));
#9987=CARTESIAN_POINT('',(0.,1.5,0.));
#9988=CARTESIAN_POINT('',(-8.73030399291527,1.5,5.));
#9989=CARTESIAN_POINT('',(-8.73030399291527,1.5,5.));
#9990=CARTESIAN_POINT('',(0.,1.5,5.));
#9991=CARTESIAN_POINT('Origin',(13.5,-1.65327317884893E-15,5.));
#9992=CARTESIAN_POINT('',(13.0833333333333,-4.98260864295893,0.));
#9993=CARTESIAN_POINT('',(8.73030399291527,-1.5,0.));
#9994=CARTESIAN_POINT('Origin',(13.5,-1.65327317884893E-15,0.));
#9995=CARTESIAN_POINT('',(13.0833333333333,-4.98260864295893,5.));
#9996=CARTESIAN_POINT('',(13.0833333333333,-4.98260864295893,5.));
#9997=CARTESIAN_POINT('',(8.73030399291527,-1.5,5.));
#9998=CARTESIAN_POINT('Origin',(13.5,-1.65327317884893E-15,5.));
#9999=CARTESIAN_POINT('',(8.73030399291527,-1.5,5.));
#10000=CARTESIAN_POINT('Origin',(0.,0.,5.));
#10001=CARTESIAN_POINT('',(-13.0833333333333,-4.98260864295891,0.));
#10002=CARTESIAN_POINT('Origin',(0.,0.,0.));
#10003=CARTESIAN_POINT('',(-13.0833333333333,-4.98260864295891,5.));
#10004=CARTESIAN_POINT('',(-13.0833333333333,-4.98260864295891,5.));
#10005=CARTESIAN_POINT('Origin',(0.,0.,5.));
#10006=CARTESIAN_POINT('Origin',(-13.5,-1.65327317884893E-15,5.));
#10007=CARTESIAN_POINT('',(-8.73030399291527,-1.5,0.));
#10008=CARTESIAN_POINT('Origin',(-13.5,-1.65327317884893E-15,0.));
#10009=CARTESIAN_POINT('',(-8.73030399291527,-1.5,5.));
#10010=CARTESIAN_POINT('',(-8.73030399291527,-1.5,5.));
#10011=CARTESIAN_POINT('Origin',(-13.5,-1.65327317884893E-15,5.));
#10012=CARTESIAN_POINT('Origin',(-20.5,-2.6342097227796E-15,5.));
#10013=CARTESIAN_POINT('',(-20.5,12.4,5.));
#10014=CARTESIAN_POINT('',(-20.5,-2.6342097227796E-15,5.));
#10015=CARTESIAN_POINT('',(-20.5,12.4,0.));
#10016=CARTESIAN_POINT('',(-20.5,12.4,5.));
#10017=CARTESIAN_POINT('',(-20.5,-2.6342097227796E-15,0.));
#10018=CARTESIAN_POINT('Origin',(-13.5,-1.65327317884893E-15,5.));
#10019=CARTESIAN_POINT('Origin',(-13.5,-1.65327317884893E-15,0.));
#10020=CARTESIAN_POINT('Origin',(-13.5,-1.65327317884893E-15,5.));
#10021=CARTESIAN_POINT('Origin',(0.,-1.5,5.));
#10022=CARTESIAN_POINT('',(0.,-1.5,0.));
#10023=CARTESIAN_POINT('',(0.,-1.5,5.));
#10024=CARTESIAN_POINT('Origin',(0.,0.,5.));
#10025=CARTESIAN_POINT('Origin',(8.5,12.4,5.));
#10026=CARTESIAN_POINT('Origin',(-8.5,12.4,5.));
#10027=CARTESIAN_POINT('Origin',(0.,0.,0.));
#10028=CARTESIAN_POINT('Origin',(8.5,12.4,0.));
#10029=CARTESIAN_POINT('Origin',(-8.5,12.4,0.));
#10030=CARTESIAN_POINT('Origin',(8.5,12.4,5.));
#10031=CARTESIAN_POINT('Origin',(-8.5,12.4,5.));
#11913=UNCERTAINTY_MEASURE_WITH_UNIT(LENGTH_MEASURE(0.01),#11934,
'DISTANCE_ACCURACY_VALUE',
'Maximum model space distance between geometric entities at asserted c
onnectivities');
#11922=UNCERTAINTY_MEASURE_WITH_UNIT(LENGTH_MEASURE(0.01),#11934,
'DISTANCE_ACCURACY_VALUE',
'Maximum model space distance between geometric entities at asserted c
onnectivities');
#11924=(
GEOMETRIC_REPRESENTATION_CONTEXT(3)
GLOBAL_UNCERTAINTY_ASSIGNED_CONTEXT((#11913))
GLOBAL_UNIT_ASSIGNED_CONTEXT((#11934,#11936,#11937))
REPRESENTATION_CONTEXT('','3D')
);
#11933=(
GEOMETRIC_REPRESENTATION_CONTEXT(3)
GLOBAL_UNCERTAINTY_ASSIGNED_CONTEXT((#11922))
GLOBAL_UNIT_ASSIGNED_CONTEXT((#11934,#11936,#11937))
REPRESENTATION_CONTEXT('','3D')
);
#11934=(
LENGTH_UNIT()
NAMED_UNIT(*)
SI_UNIT(.MILLI.,.METRE.)
);
#11936=(
NAMED_UNIT(*)
PLANE_ANGLE_UNIT()
SI_UNIT($,.RADIAN.)
);
#11937=(
NAMED_UNIT(*)
SI_UNIT($,.STERADIAN.)
SOLID_ANGLE_UNIT()
);
#11939=SHAPE_DEFINITION_REPRESENTATION(#11949,#11988);
#11949=PRODUCT_DEFINITION_SHAPE('',$,#11999);
#11988=SHAPE_REPRESENTATION('',(#6753),#11924);
#11997=PRODUCT_DEFINITION_CONTEXT('part definition',#12029,'design');
#11999=PRODUCT_DEFINITION('Mounting plate','Mounting Plate',#12009,#11997);
#12009=PRODUCT_DEFINITION_FORMATION('',$,#12032);
#12029=APPLICATION_CONTEXT(
'Core Data for Automotive Mechanical Design Process');
#12030=PRODUCT_CONTEXT('part definition',#12029,'mechanical');
#12032=PRODUCT('Mounting plate','Mounting Plate','Mounting plate',(#12030));
#12042=PRESENTATION_STYLE_ASSIGNMENT((#12046));
#12046=SURFACE_STYLE_USAGE(.BOTH.,#12050);
#12050=SURFACE_SIDE_STYLE('',(#12054));
#12054=SURFACE_STYLE_FILL_AREA(#12058);
#12058=FILL_AREA_STYLE('Opaque(227,224,212)',(#12062));
#12062=FILL_AREA_STYLE_COLOUR('Opaque(227,224,212)',#12066);
#12066=COLOUR_RGB('Opaque(227,224,212)',0.890196078431372,0.87843137254902,
0.831372549019608);
ENDSEC;
END-ISO-10303-21;
